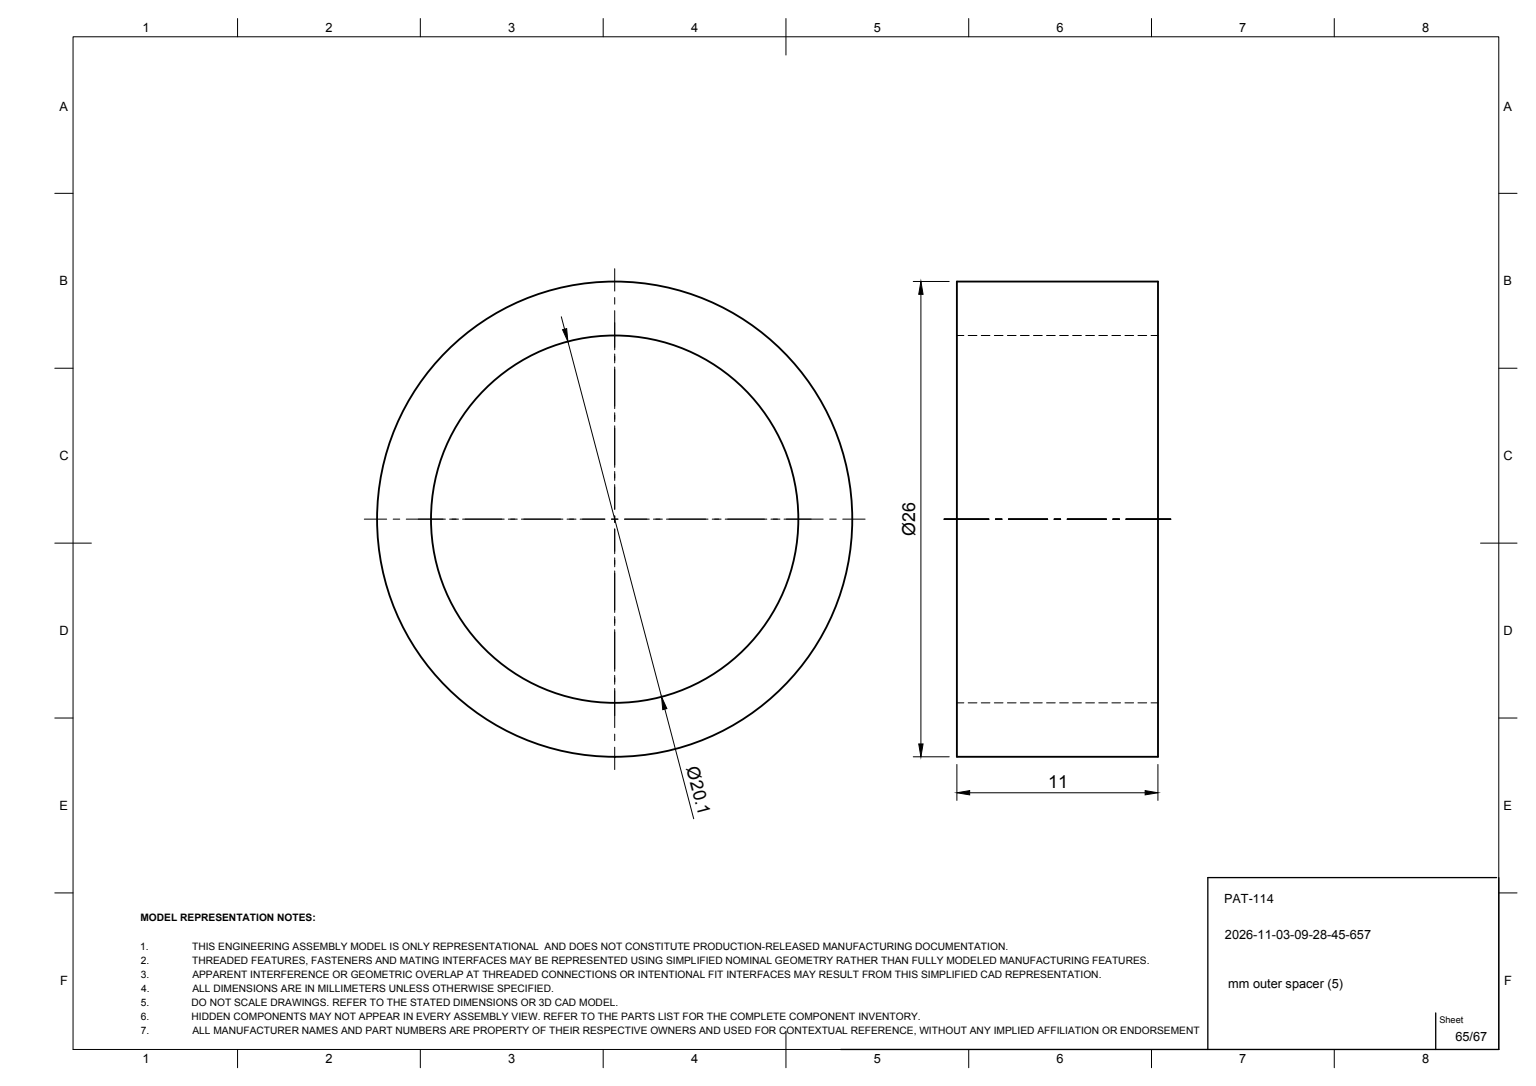
ISO-10303-21;
HEADER;
/* Generated by software containing ST-Developer
 * from STEP Tools, Inc. (www.steptools.com) 
 */

FILE_DESCRIPTION(
/* description */ ('Two-stage gear reducer in split housing'),
/* implementation_level */ '2;1');

FILE_NAME(
/* name */ 'mm outer spacer (5).step',
/* time_stamp */ '2026-10-28T03:22:31-07:00',
/* author */ (''),
/* organization */ (''),
/* preprocessor_version */ 'ST-DEVELOPER v20.2',
/* originating_system */ 'Autodesk Translation Framework v15.17.0.0',
/* authorisation */ '');

FILE_SCHEMA (('AUTOMOTIVE_DESIGN { 1 0 10303 214 3 1 1 }'));
ENDSEC;

DATA;
#10=MECHANICAL_DESIGN_GEOMETRIC_PRESENTATION_REPRESENTATION('',(#1299),#73366);
#1172=SHAPE_REPRESENTATION_RELATIONSHIP('SRR','None',#73664,#1228);
#1228=ADVANCED_BREP_SHAPE_REPRESENTATION('',(#1368),#73360);
#1299=STYLED_ITEM('',(#73974),#1368);
#1368=MANIFOLD_SOLID_BREP('Body1',#16189);
#1592=FACE_BOUND('',#3847,.T.);
#1593=FACE_BOUND('',#3849,.T.);
#1931=PLANE('',#18197);
#1932=PLANE('',#18198);
#2713=FACE_OUTER_BOUND('',#3844,.T.);
#2714=FACE_OUTER_BOUND('',#3845,.T.);
#2715=FACE_OUTER_BOUND('',#3846,.T.);
#2716=FACE_OUTER_BOUND('',#3848,.T.);
#3844=EDGE_LOOP('',(#13783,#13784,#13785,#13786));
#3845=EDGE_LOOP('',(#13787,#13788,#13789,#13790));
#3846=EDGE_LOOP('',(#13791));
#3847=EDGE_LOOP('',(#13792));
#3848=EDGE_LOOP('',(#13793));
#3849=EDGE_LOOP('',(#13794));
#4858=LINE('',#49500,#5882);
#4859=LINE('',#49506,#5883);
#5882=VECTOR('',#22022,1.005);
#5883=VECTOR('',#22029,1.3);
#6724=CIRCLE('',#18192,1.005);
#6725=CIRCLE('',#18193,1.005);
#6726=CIRCLE('',#18195,1.3);
#6727=CIRCLE('',#18196,1.3);
#7933=VERTEX_POINT('',#49497);
#7934=VERTEX_POINT('',#49499);
#7935=VERTEX_POINT('',#49503);
#7936=VERTEX_POINT('',#49505);
#9945=EDGE_CURVE('',#7933,#7933,#6724,.T.);
#9946=EDGE_CURVE('',#7933,#7934,#4858,.T.);
#9947=EDGE_CURVE('',#7934,#7934,#6725,.T.);
#9948=EDGE_CURVE('',#7935,#7935,#6726,.T.);
#9949=EDGE_CURVE('',#7935,#7936,#4859,.T.);
#9950=EDGE_CURVE('',#7936,#7936,#6727,.T.);
#13783=ORIENTED_EDGE('',*,*,#9945,.F.);
#13784=ORIENTED_EDGE('',*,*,#9946,.T.);
#13785=ORIENTED_EDGE('',*,*,#9947,.T.);
#13786=ORIENTED_EDGE('',*,*,#9946,.F.);
#13787=ORIENTED_EDGE('',*,*,#9948,.F.);
#13788=ORIENTED_EDGE('',*,*,#9949,.T.);
#13789=ORIENTED_EDGE('',*,*,#9950,.T.);
#13790=ORIENTED_EDGE('',*,*,#9949,.F.);
#13791=ORIENTED_EDGE('',*,*,#9948,.T.);
#13792=ORIENTED_EDGE('',*,*,#9945,.T.);
#13793=ORIENTED_EDGE('',*,*,#9950,.F.);
#13794=ORIENTED_EDGE('',*,*,#9947,.F.);
#15160=CYLINDRICAL_SURFACE('',#18191,1.005);
#15161=CYLINDRICAL_SURFACE('',#18194,1.3);
#15920=ADVANCED_FACE('',(#2713),#15160,.F.);
#15921=ADVANCED_FACE('',(#2714),#15161,.T.);
#15922=ADVANCED_FACE('',(#2715,#1592),#1931,.T.);
#15923=ADVANCED_FACE('',(#2716,#1593),#1932,.F.);
#16189=CLOSED_SHELL('',(#15920,#15921,#15922,#15923));
#18190=AXIS2_PLACEMENT_3D('',#49495,#22016,#22017);
#18191=AXIS2_PLACEMENT_3D('',#49496,#22018,#22019);
#18192=AXIS2_PLACEMENT_3D('',#49498,#22020,#22021);
#18193=AXIS2_PLACEMENT_3D('',#49501,#22023,#22024);
#18194=AXIS2_PLACEMENT_3D('',#49502,#22025,#22026);
#18195=AXIS2_PLACEMENT_3D('',#49504,#22027,#22028);
#18196=AXIS2_PLACEMENT_3D('',#49507,#22030,#22031);
#18197=AXIS2_PLACEMENT_3D('',#49508,#22032,#22033);
#18198=AXIS2_PLACEMENT_3D('',#49509,#22034,#22035);
#22016=DIRECTION('axis',(0.,0.,1.));
#22017=DIRECTION('refdir',(1.,0.,0.));
#22018=DIRECTION('center_axis',(0.,1.,0.));
#22019=DIRECTION('ref_axis',(1.,0.,0.));
#22020=DIRECTION('center_axis',(0.,-1.,0.));
#22021=DIRECTION('ref_axis',(1.,0.,0.));
#22022=DIRECTION('',(0.,-1.,0.));
#22023=DIRECTION('center_axis',(0.,-1.,0.));
#22024=DIRECTION('ref_axis',(1.,0.,0.));
#22025=DIRECTION('center_axis',(0.,1.,0.));
#22026=DIRECTION('ref_axis',(1.,0.,0.));
#22027=DIRECTION('center_axis',(0.,1.,0.));
#22028=DIRECTION('ref_axis',(1.,0.,0.));
#22029=DIRECTION('',(0.,-1.,0.));
#22030=DIRECTION('center_axis',(0.,1.,0.));
#22031=DIRECTION('ref_axis',(1.,0.,0.));
#22032=DIRECTION('center_axis',(0.,1.,0.));
#22033=DIRECTION('ref_axis',(1.,0.,0.));
#22034=DIRECTION('center_axis',(0.,1.,0.));
#22035=DIRECTION('ref_axis',(1.,0.,0.));
#49495=CARTESIAN_POINT('',(0.,0.,0.));
#49496=CARTESIAN_POINT('Origin',(12.,6.7,10.));
#49497=CARTESIAN_POINT('',(10.995,7.8,10.));
#49498=CARTESIAN_POINT('Origin',(12.,7.8,10.));
#49499=CARTESIAN_POINT('',(10.995,6.7,10.));
#49500=CARTESIAN_POINT('',(10.995,6.7,10.));
#49501=CARTESIAN_POINT('Origin',(12.,6.7,10.));
#49502=CARTESIAN_POINT('Origin',(12.,6.7,10.));
#49503=CARTESIAN_POINT('',(10.7,7.8,10.));
#49504=CARTESIAN_POINT('Origin',(12.,7.8,10.));
#49505=CARTESIAN_POINT('',(10.7,6.7,10.));
#49506=CARTESIAN_POINT('',(10.7,6.7,10.));
#49507=CARTESIAN_POINT('Origin',(12.,6.7,10.));
#49508=CARTESIAN_POINT('Origin',(12.,7.8,10.));
#49509=CARTESIAN_POINT('Origin',(12.,6.7,10.));
#73296=UNCERTAINTY_MEASURE_WITH_UNIT(LENGTH_MEASURE(0.001),#73367,
'DISTANCE_ACCURACY_VALUE',
'Maximum model space distance between geometric entities at asserted c
onnectivities');
#73302=UNCERTAINTY_MEASURE_WITH_UNIT(LENGTH_MEASURE(0.001),#73367,
'DISTANCE_ACCURACY_VALUE',
'Maximum model space distance between geometric entities at asserted c
onnectivities');
#73360=(
GEOMETRIC_REPRESENTATION_CONTEXT(3)
GLOBAL_UNCERTAINTY_ASSIGNED_CONTEXT((#73296))
GLOBAL_UNIT_ASSIGNED_CONTEXT((#73367,#73369,#73370))
REPRESENTATION_CONTEXT('','3D')
);
#73366=(
GEOMETRIC_REPRESENTATION_CONTEXT(3)
GLOBAL_UNCERTAINTY_ASSIGNED_CONTEXT((#73302))
GLOBAL_UNIT_ASSIGNED_CONTEXT((#73367,#73369,#73370))
REPRESENTATION_CONTEXT('','3D')
);
#73367=(
LENGTH_UNIT()
NAMED_UNIT(*)
SI_UNIT(.CENTI.,.METRE.)
);
#73369=(
NAMED_UNIT(*)
PLANE_ANGLE_UNIT()
SI_UNIT($,.RADIAN.)
);
#73370=(
NAMED_UNIT(*)
SI_UNIT($,.STERADIAN.)
SOLID_ANGLE_UNIT()
);
#73428=SHAPE_DEFINITION_REPRESENTATION(#73561,#73664);
#73561=PRODUCT_DEFINITION_SHAPE('',$,#73728);
#73664=SHAPE_REPRESENTATION('',(#18190),#73360);
#73670=PRODUCT_DEFINITION_CONTEXT('part definition',#73861,'design');
#73728=PRODUCT_DEFINITION('mm outer spacer (5)','mm outer spacer (5)',#73791,
#73670);
#73791=PRODUCT_DEFINITION_FORMATION('',$,#73920);
#73861=APPLICATION_CONTEXT(
'Core Data for Automotive Mechanical Design Process');
#73862=PRODUCT_CONTEXT('part definition',#73861,'mechanical');
#73920=PRODUCT('mm outer spacer (5)','mm outer spacer (5)',
'mm outer spacer (5)',(#73862));
#73968=COLOUR_RGB('Light Blue',0.38,0.62,0.78);
#73969=FILL_AREA_STYLE_COLOUR('',#73968);
#73970=FILL_AREA_STYLE('',(#73969));
#73971=SURFACE_STYLE_FILL_AREA(#73970);
#73972=SURFACE_SIDE_STYLE('',(#73971));
#73973=SURFACE_STYLE_USAGE(.BOTH.,#73972);
#73974=PRESENTATION_STYLE_ASSIGNMENT((#73973));
ENDSEC;
END-ISO-10303-21;
